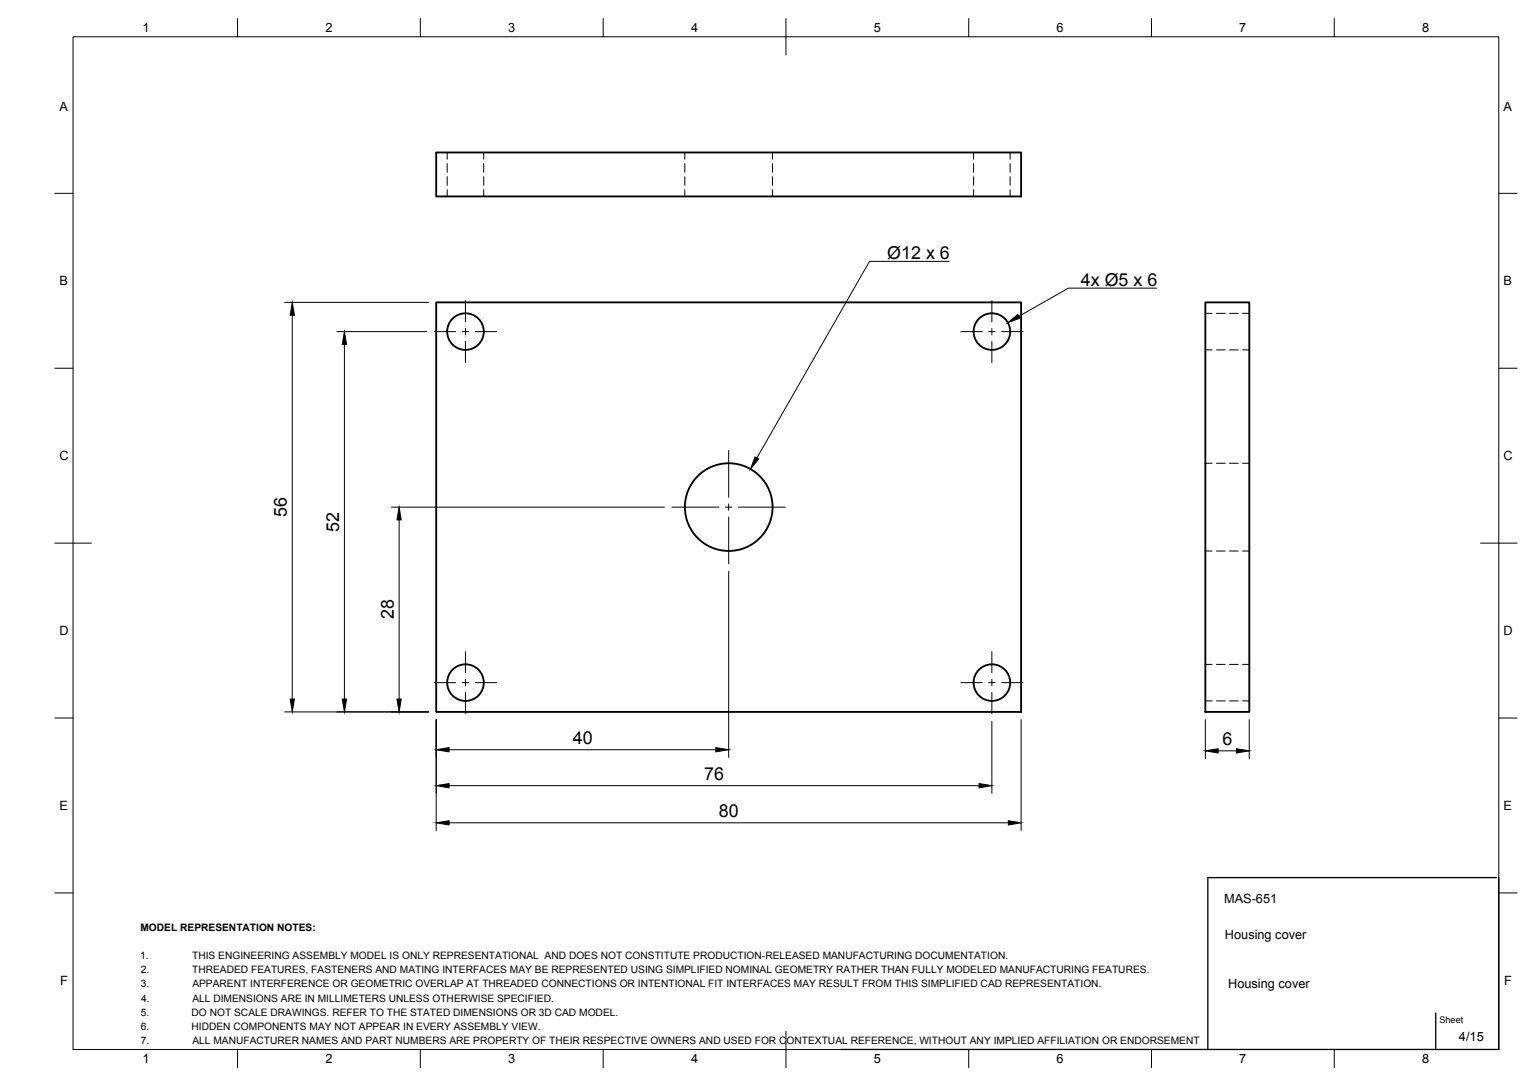
ISO-10303-21;
HEADER;
/* Generated by software containing ST-Developer
 * from STEP Tools, Inc. (www.steptools.com) 
 */

FILE_DESCRIPTION(
/* description */ ('Independent direct-acting normally-closed roller-plunger limit-switch
 CAD. Removable cover, insulated terminal supports, captured bus/conta
ct bridge, native Coil return spring, integral lower travel stop, reus
able instanced hardware and free roller. Manual geometric contact open
ing4mm; no snap-action/contact-force, electrical/current/voltage, envi
ronmental seal, safety-switch, wear, load or life certification. Exter
nal wiring and anchors omitted; fits and application engineering requi
red.'),
/* implementation_level */ '2;1');

FILE_NAME(
/* name */ 'Housing cover.step',
/* time_stamp */ '2026-11-08T07:32:43-08:00',
/* author */ (''),
/* organization */ (''),
/* preprocessor_version */ 'ST-DEVELOPER v20.2',
/* originating_system */ 'Autodesk Translation Framework v15.17.0.0',
/* authorisation */ '');

FILE_SCHEMA (('AUTOMOTIVE_DESIGN { 1 0 10303 214 3 1 1 }'));
ENDSEC;

DATA;
#10=MECHANICAL_DESIGN_GEOMETRIC_PRESENTATION_REPRESENTATION('',(#177),#36482);
#143=SHAPE_REPRESENTATION_RELATIONSHIP('SRR','None',#36556,#160);
#160=ADVANCED_BREP_SHAPE_REPRESENTATION('',(#194),#36466);
#177=STYLED_ITEM('',(#36650),#194);
#194=MANIFOLD_SOLID_BREP('Body1',#9768);
#254=FACE_BOUND('',#1166,.T.);
#255=FACE_BOUND('',#1167,.T.);
#256=FACE_BOUND('',#1168,.T.);
#257=FACE_BOUND('',#1169,.T.);
#258=FACE_BOUND('',#1170,.T.);
#259=FACE_BOUND('',#1172,.T.);
#260=FACE_BOUND('',#1173,.T.);
#261=FACE_BOUND('',#1174,.T.);
#262=FACE_BOUND('',#1175,.T.);
#263=FACE_BOUND('',#1176,.T.);
#333=PLANE('',#10188);
#334=PLANE('',#10189);
#335=PLANE('',#10190);
#336=PLANE('',#10191);
#337=PLANE('',#10192);
#338=PLANE('',#10193);
#599=FACE_OUTER_BOUND('',#1156,.T.);
#600=FACE_OUTER_BOUND('',#1157,.T.);
#601=FACE_OUTER_BOUND('',#1158,.T.);
#602=FACE_OUTER_BOUND('',#1159,.T.);
#603=FACE_OUTER_BOUND('',#1160,.T.);
#604=FACE_OUTER_BOUND('',#1161,.T.);
#605=FACE_OUTER_BOUND('',#1162,.T.);
#606=FACE_OUTER_BOUND('',#1163,.T.);
#607=FACE_OUTER_BOUND('',#1164,.T.);
#608=FACE_OUTER_BOUND('',#1165,.T.);
#609=FACE_OUTER_BOUND('',#1171,.T.);
#1156=EDGE_LOOP('',(#6880,#6881,#6882,#6883));
#1157=EDGE_LOOP('',(#6884,#6885,#6886,#6887));
#1158=EDGE_LOOP('',(#6888,#6889,#6890,#6891));
#1159=EDGE_LOOP('',(#6892,#6893,#6894,#6895));
#1160=EDGE_LOOP('',(#6896,#6897,#6898,#6899));
#1161=EDGE_LOOP('',(#6900,#6901,#6902,#6903));
#1162=EDGE_LOOP('',(#6904,#6905,#6906,#6907));
#1163=EDGE_LOOP('',(#6908,#6909,#6910,#6911));
#1164=EDGE_LOOP('',(#6912,#6913,#6914,#6915));
#1165=EDGE_LOOP('',(#6916,#6917,#6918,#6919));
#1166=EDGE_LOOP('',(#6920));
#1167=EDGE_LOOP('',(#6921));
#1168=EDGE_LOOP('',(#6922));
#1169=EDGE_LOOP('',(#6923));
#1170=EDGE_LOOP('',(#6924));
#1171=EDGE_LOOP('',(#6925,#6926,#6927,#6928));
#1172=EDGE_LOOP('',(#6929));
#1173=EDGE_LOOP('',(#6930));
#1174=EDGE_LOOP('',(#6931));
#1175=EDGE_LOOP('',(#6932));
#1176=EDGE_LOOP('',(#6933));
#1628=CIRCLE('',#10174,0.25);
#1629=CIRCLE('',#10175,0.25);
#1630=CIRCLE('',#10177,0.25);
#1631=CIRCLE('',#10178,0.25);
#1632=CIRCLE('',#10180,0.25);
#1633=CIRCLE('',#10181,0.25);
#1634=CIRCLE('',#10183,0.25);
#1635=CIRCLE('',#10184,0.25);
#1636=CIRCLE('',#10186,0.6);
#1637=CIRCLE('',#10187,0.6);
#2610=LINE('',#20404,#3184);
#2611=LINE('',#20410,#3185);
#2612=LINE('',#20416,#3186);
#2613=LINE('',#20422,#3187);
#2614=LINE('',#20428,#3188);
#2615=LINE('',#20433,#3189);
#2616=LINE('',#20435,#3190);
#2617=LINE('',#20437,#3191);
#2618=LINE('',#20438,#3192);
#2619=LINE('',#20441,#3193);
#2620=LINE('',#20443,#3194);
#2621=LINE('',#20444,#3195);
#2622=LINE('',#20447,#3196);
#2623=LINE('',#20449,#3197);
#2624=LINE('',#20450,#3198);
#2625=LINE('',#20452,#3199);
#2626=LINE('',#20453,#3200);
#3184=VECTOR('',#11261,0.25);
#3185=VECTOR('',#11268,0.25);
#3186=VECTOR('',#11275,0.25);
#3187=VECTOR('',#11282,0.25);
#3188=VECTOR('',#11289,0.6);
#3189=VECTOR('',#11294,1.);
#3190=VECTOR('',#11295,1.);
#3191=VECTOR('',#11296,1.);
#3192=VECTOR('',#11297,1.);
#3193=VECTOR('',#11300,1.);
#3194=VECTOR('',#11301,1.);
#3195=VECTOR('',#11302,1.);
#3196=VECTOR('',#11305,1.);
#3197=VECTOR('',#11306,1.);
#3198=VECTOR('',#11307,1.);
#3199=VECTOR('',#11310,1.);
#3200=VECTOR('',#11311,1.);
#3891=VERTEX_POINT('',#20401);
#3892=VERTEX_POINT('',#20403);
#3893=VERTEX_POINT('',#20407);
#3894=VERTEX_POINT('',#20409);
#3895=VERTEX_POINT('',#20413);
#3896=VERTEX_POINT('',#20415);
#3897=VERTEX_POINT('',#20419);
#3898=VERTEX_POINT('',#20421);
#3899=VERTEX_POINT('',#20425);
#3900=VERTEX_POINT('',#20427);
#3901=VERTEX_POINT('',#20431);
#3902=VERTEX_POINT('',#20432);
#3903=VERTEX_POINT('',#20434);
#3904=VERTEX_POINT('',#20436);
#3905=VERTEX_POINT('',#20440);
#3906=VERTEX_POINT('',#20442);
#3907=VERTEX_POINT('',#20446);
#3908=VERTEX_POINT('',#20448);
#4996=EDGE_CURVE('',#3891,#3891,#1628,.T.);
#4997=EDGE_CURVE('',#3891,#3892,#2610,.T.);
#4998=EDGE_CURVE('',#3892,#3892,#1629,.T.);
#4999=EDGE_CURVE('',#3893,#3893,#1630,.T.);
#5000=EDGE_CURVE('',#3893,#3894,#2611,.T.);
#5001=EDGE_CURVE('',#3894,#3894,#1631,.T.);
#5002=EDGE_CURVE('',#3895,#3895,#1632,.T.);
#5003=EDGE_CURVE('',#3895,#3896,#2612,.T.);
#5004=EDGE_CURVE('',#3896,#3896,#1633,.T.);
#5005=EDGE_CURVE('',#3897,#3897,#1634,.T.);
#5006=EDGE_CURVE('',#3897,#3898,#2613,.T.);
#5007=EDGE_CURVE('',#3898,#3898,#1635,.T.);
#5008=EDGE_CURVE('',#3899,#3899,#1636,.T.);
#5009=EDGE_CURVE('',#3899,#3900,#2614,.T.);
#5010=EDGE_CURVE('',#3900,#3900,#1637,.T.);
#5011=EDGE_CURVE('',#3901,#3902,#2615,.T.);
#5012=EDGE_CURVE('',#3902,#3903,#2616,.T.);
#5013=EDGE_CURVE('',#3904,#3903,#2617,.T.);
#5014=EDGE_CURVE('',#3901,#3904,#2618,.T.);
#5015=EDGE_CURVE('',#3905,#3901,#2619,.T.);
#5016=EDGE_CURVE('',#3906,#3904,#2620,.T.);
#5017=EDGE_CURVE('',#3905,#3906,#2621,.T.);
#5018=EDGE_CURVE('',#3907,#3905,#2622,.T.);
#5019=EDGE_CURVE('',#3908,#3906,#2623,.T.);
#5020=EDGE_CURVE('',#3907,#3908,#2624,.T.);
#5021=EDGE_CURVE('',#3902,#3907,#2625,.T.);
#5022=EDGE_CURVE('',#3903,#3908,#2626,.T.);
#6880=ORIENTED_EDGE('',*,*,#4996,.F.);
#6881=ORIENTED_EDGE('',*,*,#4997,.T.);
#6882=ORIENTED_EDGE('',*,*,#4998,.F.);
#6883=ORIENTED_EDGE('',*,*,#4997,.F.);
#6884=ORIENTED_EDGE('',*,*,#4999,.F.);
#6885=ORIENTED_EDGE('',*,*,#5000,.T.);
#6886=ORIENTED_EDGE('',*,*,#5001,.F.);
#6887=ORIENTED_EDGE('',*,*,#5000,.F.);
#6888=ORIENTED_EDGE('',*,*,#5002,.F.);
#6889=ORIENTED_EDGE('',*,*,#5003,.T.);
#6890=ORIENTED_EDGE('',*,*,#5004,.F.);
#6891=ORIENTED_EDGE('',*,*,#5003,.F.);
#6892=ORIENTED_EDGE('',*,*,#5005,.F.);
#6893=ORIENTED_EDGE('',*,*,#5006,.T.);
#6894=ORIENTED_EDGE('',*,*,#5007,.F.);
#6895=ORIENTED_EDGE('',*,*,#5006,.F.);
#6896=ORIENTED_EDGE('',*,*,#5008,.F.);
#6897=ORIENTED_EDGE('',*,*,#5009,.T.);
#6898=ORIENTED_EDGE('',*,*,#5010,.F.);
#6899=ORIENTED_EDGE('',*,*,#5009,.F.);
#6900=ORIENTED_EDGE('',*,*,#5011,.T.);
#6901=ORIENTED_EDGE('',*,*,#5012,.T.);
#6902=ORIENTED_EDGE('',*,*,#5013,.F.);
#6903=ORIENTED_EDGE('',*,*,#5014,.F.);
#6904=ORIENTED_EDGE('',*,*,#5015,.T.);
#6905=ORIENTED_EDGE('',*,*,#5014,.T.);
#6906=ORIENTED_EDGE('',*,*,#5016,.F.);
#6907=ORIENTED_EDGE('',*,*,#5017,.F.);
#6908=ORIENTED_EDGE('',*,*,#5018,.T.);
#6909=ORIENTED_EDGE('',*,*,#5017,.T.);
#6910=ORIENTED_EDGE('',*,*,#5019,.F.);
#6911=ORIENTED_EDGE('',*,*,#5020,.F.);
#6912=ORIENTED_EDGE('',*,*,#5021,.T.);
#6913=ORIENTED_EDGE('',*,*,#5020,.T.);
#6914=ORIENTED_EDGE('',*,*,#5022,.F.);
#6915=ORIENTED_EDGE('',*,*,#5012,.F.);
#6916=ORIENTED_EDGE('',*,*,#5022,.T.);
#6917=ORIENTED_EDGE('',*,*,#5019,.T.);
#6918=ORIENTED_EDGE('',*,*,#5016,.T.);
#6919=ORIENTED_EDGE('',*,*,#5013,.T.);
#6920=ORIENTED_EDGE('',*,*,#5008,.T.);
#6921=ORIENTED_EDGE('',*,*,#5005,.T.);
#6922=ORIENTED_EDGE('',*,*,#5002,.T.);
#6923=ORIENTED_EDGE('',*,*,#4999,.T.);
#6924=ORIENTED_EDGE('',*,*,#4996,.T.);
#6925=ORIENTED_EDGE('',*,*,#5021,.F.);
#6926=ORIENTED_EDGE('',*,*,#5011,.F.);
#6927=ORIENTED_EDGE('',*,*,#5015,.F.);
#6928=ORIENTED_EDGE('',*,*,#5018,.F.);
#6929=ORIENTED_EDGE('',*,*,#5010,.T.);
#6930=ORIENTED_EDGE('',*,*,#5007,.T.);
#6931=ORIENTED_EDGE('',*,*,#5004,.T.);
#6932=ORIENTED_EDGE('',*,*,#5001,.T.);
#6933=ORIENTED_EDGE('',*,*,#4998,.T.);
#8981=CYLINDRICAL_SURFACE('',#10173,0.25);
#8982=CYLINDRICAL_SURFACE('',#10176,0.25);
#8983=CYLINDRICAL_SURFACE('',#10179,0.25);
#8984=CYLINDRICAL_SURFACE('',#10182,0.25);
#8985=CYLINDRICAL_SURFACE('',#10185,0.6);
#9389=ADVANCED_FACE('',(#599),#8981,.F.);
#9390=ADVANCED_FACE('',(#600),#8982,.F.);
#9391=ADVANCED_FACE('',(#601),#8983,.F.);
#9392=ADVANCED_FACE('',(#602),#8984,.F.);
#9393=ADVANCED_FACE('',(#603),#8985,.F.);
#9394=ADVANCED_FACE('',(#604),#333,.T.);
#9395=ADVANCED_FACE('',(#605),#334,.T.);
#9396=ADVANCED_FACE('',(#606),#335,.T.);
#9397=ADVANCED_FACE('',(#607),#336,.T.);
#9398=ADVANCED_FACE('',(#608,#254,#255,#256,#257,#258),#337,.T.);
#9399=ADVANCED_FACE('',(#609,#259,#260,#261,#262,#263),#338,.F.);
#9768=CLOSED_SHELL('',(#9389,#9390,#9391,#9392,#9393,#9394,#9395,#9396,
#9397,#9398,#9399));
#10172=AXIS2_PLACEMENT_3D('',#20399,#11255,#11256);
#10173=AXIS2_PLACEMENT_3D('',#20400,#11257,#11258);
#10174=AXIS2_PLACEMENT_3D('',#20402,#11259,#11260);
#10175=AXIS2_PLACEMENT_3D('',#20405,#11262,#11263);
#10176=AXIS2_PLACEMENT_3D('',#20406,#11264,#11265);
#10177=AXIS2_PLACEMENT_3D('',#20408,#11266,#11267);
#10178=AXIS2_PLACEMENT_3D('',#20411,#11269,#11270);
#10179=AXIS2_PLACEMENT_3D('',#20412,#11271,#11272);
#10180=AXIS2_PLACEMENT_3D('',#20414,#11273,#11274);
#10181=AXIS2_PLACEMENT_3D('',#20417,#11276,#11277);
#10182=AXIS2_PLACEMENT_3D('',#20418,#11278,#11279);
#10183=AXIS2_PLACEMENT_3D('',#20420,#11280,#11281);
#10184=AXIS2_PLACEMENT_3D('',#20423,#11283,#11284);
#10185=AXIS2_PLACEMENT_3D('',#20424,#11285,#11286);
#10186=AXIS2_PLACEMENT_3D('',#20426,#11287,#11288);
#10187=AXIS2_PLACEMENT_3D('',#20429,#11290,#11291);
#10188=AXIS2_PLACEMENT_3D('',#20430,#11292,#11293);
#10189=AXIS2_PLACEMENT_3D('',#20439,#11298,#11299);
#10190=AXIS2_PLACEMENT_3D('',#20445,#11303,#11304);
#10191=AXIS2_PLACEMENT_3D('',#20451,#11308,#11309);
#10192=AXIS2_PLACEMENT_3D('',#20454,#11312,#11313);
#10193=AXIS2_PLACEMENT_3D('',#20455,#11314,#11315);
#11255=DIRECTION('axis',(0.,0.,1.));
#11256=DIRECTION('refdir',(1.,0.,0.));
#11257=DIRECTION('center_axis',(0.,0.,-1.));
#11258=DIRECTION('ref_axis',(1.,0.,0.));
#11259=DIRECTION('center_axis',(0.,0.,-1.));
#11260=DIRECTION('ref_axis',(1.,0.,0.));
#11261=DIRECTION('',(0.,0.,-1.));
#11262=DIRECTION('center_axis',(0.,0.,1.));
#11263=DIRECTION('ref_axis',(1.,0.,0.));
#11264=DIRECTION('center_axis',(0.,0.,-1.));
#11265=DIRECTION('ref_axis',(1.,0.,0.));
#11266=DIRECTION('center_axis',(0.,0.,-1.));
#11267=DIRECTION('ref_axis',(1.,0.,0.));
#11268=DIRECTION('',(0.,0.,-1.));
#11269=DIRECTION('center_axis',(0.,0.,1.));
#11270=DIRECTION('ref_axis',(1.,0.,0.));
#11271=DIRECTION('center_axis',(0.,0.,-1.));
#11272=DIRECTION('ref_axis',(1.,0.,0.));
#11273=DIRECTION('center_axis',(0.,0.,-1.));
#11274=DIRECTION('ref_axis',(1.,0.,0.));
#11275=DIRECTION('',(0.,0.,-1.));
#11276=DIRECTION('center_axis',(0.,0.,1.));
#11277=DIRECTION('ref_axis',(1.,0.,0.));
#11278=DIRECTION('center_axis',(0.,0.,-1.));
#11279=DIRECTION('ref_axis',(1.,0.,0.));
#11280=DIRECTION('center_axis',(0.,0.,-1.));
#11281=DIRECTION('ref_axis',(1.,0.,0.));
#11282=DIRECTION('',(0.,0.,-1.));
#11283=DIRECTION('center_axis',(0.,0.,1.));
#11284=DIRECTION('ref_axis',(1.,0.,0.));
#11285=DIRECTION('center_axis',(0.,0.,-1.));
#11286=DIRECTION('ref_axis',(1.,0.,0.));
#11287=DIRECTION('center_axis',(0.,0.,-1.));
#11288=DIRECTION('ref_axis',(1.,0.,0.));
#11289=DIRECTION('',(0.,0.,-1.));
#11290=DIRECTION('center_axis',(0.,0.,1.));
#11291=DIRECTION('ref_axis',(1.,0.,0.));
#11292=DIRECTION('center_axis',(0.,1.,0.));
#11293=DIRECTION('ref_axis',(-1.,0.,0.));
#11294=DIRECTION('',(-1.,0.,0.));
#11295=DIRECTION('',(0.,0.,1.));
#11296=DIRECTION('',(-1.,0.,0.));
#11297=DIRECTION('',(0.,0.,1.));
#11298=DIRECTION('center_axis',(1.,0.,0.));
#11299=DIRECTION('ref_axis',(0.,1.,0.));
#11300=DIRECTION('',(0.,1.,0.));
#11301=DIRECTION('',(0.,1.,0.));
#11302=DIRECTION('',(0.,0.,1.));
#11303=DIRECTION('center_axis',(0.,-1.,0.));
#11304=DIRECTION('ref_axis',(1.,0.,0.));
#11305=DIRECTION('',(1.,0.,0.));
#11306=DIRECTION('',(1.,0.,0.));
#11307=DIRECTION('',(0.,0.,1.));
#11308=DIRECTION('center_axis',(-1.,0.,0.));
#11309=DIRECTION('ref_axis',(0.,-1.,0.));
#11310=DIRECTION('',(0.,-1.,0.));
#11311=DIRECTION('',(0.,-1.,0.));
#11312=DIRECTION('center_axis',(0.,0.,1.));
#11313=DIRECTION('ref_axis',(1.,0.,0.));
#11314=DIRECTION('center_axis',(0.,0.,1.));
#11315=DIRECTION('ref_axis',(1.,0.,0.));
#20399=CARTESIAN_POINT('',(0.,0.,0.));
#20400=CARTESIAN_POINT('Origin',(3.6,-2.4,5.5));
#20401=CARTESIAN_POINT('',(3.35,-2.4,5.8));
#20402=CARTESIAN_POINT('Origin',(3.6,-2.4,5.8));
#20403=CARTESIAN_POINT('',(3.35,-2.4,5.2));
#20404=CARTESIAN_POINT('',(3.35,-2.4,5.5));
#20405=CARTESIAN_POINT('Origin',(3.6,-2.4,5.2));
#20406=CARTESIAN_POINT('Origin',(-3.6,-2.4,5.5));
#20407=CARTESIAN_POINT('',(-3.85,-2.4,5.8));
#20408=CARTESIAN_POINT('Origin',(-3.6,-2.4,5.8));
#20409=CARTESIAN_POINT('',(-3.85,-2.4,5.2));
#20410=CARTESIAN_POINT('',(-3.85,-2.4,5.5));
#20411=CARTESIAN_POINT('Origin',(-3.6,-2.4,5.2));
#20412=CARTESIAN_POINT('Origin',(-3.6,2.4,5.5));
#20413=CARTESIAN_POINT('',(-3.85,2.4,5.8));
#20414=CARTESIAN_POINT('Origin',(-3.6,2.4,5.8));
#20415=CARTESIAN_POINT('',(-3.85,2.4,5.2));
#20416=CARTESIAN_POINT('',(-3.85,2.4,5.5));
#20417=CARTESIAN_POINT('Origin',(-3.6,2.4,5.2));
#20418=CARTESIAN_POINT('Origin',(3.6,2.4,5.5));
#20419=CARTESIAN_POINT('',(3.35,2.4,5.8));
#20420=CARTESIAN_POINT('Origin',(3.6,2.4,5.8));
#20421=CARTESIAN_POINT('',(3.35,2.4,5.2));
#20422=CARTESIAN_POINT('',(3.35,2.4,5.5));
#20423=CARTESIAN_POINT('Origin',(3.6,2.4,5.2));
#20424=CARTESIAN_POINT('Origin',(0.,0.,5.5));
#20425=CARTESIAN_POINT('',(-0.6,7.34788079488412E-17,5.8));
#20426=CARTESIAN_POINT('Origin',(0.,0.,5.8));
#20427=CARTESIAN_POINT('',(-0.6,7.34788079488412E-17,5.2));
#20428=CARTESIAN_POINT('',(-0.6,7.34788079488412E-17,5.5));
#20429=CARTESIAN_POINT('Origin',(0.,0.,5.2));
#20430=CARTESIAN_POINT('Origin',(4.,2.8,5.2));
#20431=CARTESIAN_POINT('',(4.,2.8,5.2));
#20432=CARTESIAN_POINT('',(-4.,2.8,5.2));
#20433=CARTESIAN_POINT('',(4.,2.8,5.2));
#20434=CARTESIAN_POINT('',(-4.,2.8,5.8));
#20435=CARTESIAN_POINT('',(-4.,2.8,5.2));
#20436=CARTESIAN_POINT('',(4.,2.8,5.8));
#20437=CARTESIAN_POINT('',(4.,2.8,5.8));
#20438=CARTESIAN_POINT('',(4.,2.8,5.2));
#20439=CARTESIAN_POINT('Origin',(4.,-2.8,5.2));
#20440=CARTESIAN_POINT('',(4.,-2.8,5.2));
#20441=CARTESIAN_POINT('',(4.,-2.8,5.2));
#20442=CARTESIAN_POINT('',(4.,-2.8,5.8));
#20443=CARTESIAN_POINT('',(4.,-2.8,5.8));
#20444=CARTESIAN_POINT('',(4.,-2.8,5.2));
#20445=CARTESIAN_POINT('Origin',(-4.,-2.8,5.2));
#20446=CARTESIAN_POINT('',(-4.,-2.8,5.2));
#20447=CARTESIAN_POINT('',(-4.,-2.8,5.2));
#20448=CARTESIAN_POINT('',(-4.,-2.8,5.8));
#20449=CARTESIAN_POINT('',(-4.,-2.8,5.8));
#20450=CARTESIAN_POINT('',(-4.,-2.8,5.2));
#20451=CARTESIAN_POINT('Origin',(-4.,2.8,5.2));
#20452=CARTESIAN_POINT('',(-4.,2.8,5.2));
#20453=CARTESIAN_POINT('',(-4.,2.8,5.8));
#20454=CARTESIAN_POINT('Origin',(0.,0.,5.8));
#20455=CARTESIAN_POINT('Origin',(0.,0.,5.2));
#36447=UNCERTAINTY_MEASURE_WITH_UNIT(LENGTH_MEASURE(0.001),#36483,
'DISTANCE_ACCURACY_VALUE',
'Maximum model space distance between geometric entities at asserted c
onnectivities');
#36463=UNCERTAINTY_MEASURE_WITH_UNIT(LENGTH_MEASURE(0.001),#36483,
'DISTANCE_ACCURACY_VALUE',
'Maximum model space distance between geometric entities at asserted c
onnectivities');
#36466=(
GEOMETRIC_REPRESENTATION_CONTEXT(3)
GLOBAL_UNCERTAINTY_ASSIGNED_CONTEXT((#36447))
GLOBAL_UNIT_ASSIGNED_CONTEXT((#36483,#36485,#36486))
REPRESENTATION_CONTEXT('','3D')
);
#36482=(
GEOMETRIC_REPRESENTATION_CONTEXT(3)
GLOBAL_UNCERTAINTY_ASSIGNED_CONTEXT((#36463))
GLOBAL_UNIT_ASSIGNED_CONTEXT((#36483,#36485,#36486))
REPRESENTATION_CONTEXT('','3D')
);
#36483=(
LENGTH_UNIT()
NAMED_UNIT(*)
SI_UNIT(.CENTI.,.METRE.)
);
#36485=(
NAMED_UNIT(*)
PLANE_ANGLE_UNIT()
SI_UNIT($,.RADIAN.)
);
#36486=(
NAMED_UNIT(*)
SI_UNIT($,.STERADIAN.)
SOLID_ANGLE_UNIT()
);
#36489=SHAPE_DEFINITION_REPRESENTATION(#36507,#36556);
#36507=PRODUCT_DEFINITION_SHAPE('',$,#36575);
#36556=SHAPE_REPRESENTATION('',(#10172),#36466);
#36572=PRODUCT_DEFINITION_CONTEXT('part definition',#36628,'design');
#36575=PRODUCT_DEFINITION('Housing cover','Housing cover',#36593,#36572);
#36593=PRODUCT_DEFINITION_FORMATION('',$,#36632);
#36628=APPLICATION_CONTEXT(
'Core Data for Automotive Mechanical Design Process');
#36629=PRODUCT_CONTEXT('part definition',#36628,'mechanical');
#36632=PRODUCT('Housing cover','Housing cover',$,(#36629));
#36650=PRESENTATION_STYLE_ASSIGNMENT((#36664));
#36664=SURFACE_STYLE_USAGE(.BOTH.,#36678);
#36678=SURFACE_SIDE_STYLE('',(#36692));
#36692=SURFACE_STYLE_FILL_AREA(#36706);
#36706=FILL_AREA_STYLE('Sky blue',(#36720));
#36720=FILL_AREA_STYLE_COLOUR('Sky blue',#36734);
#36734=COLOUR_RGB('Sky blue',0.317647058823529,0.686274509803922,0.890196078431372);
ENDSEC;
END-ISO-10303-21;
